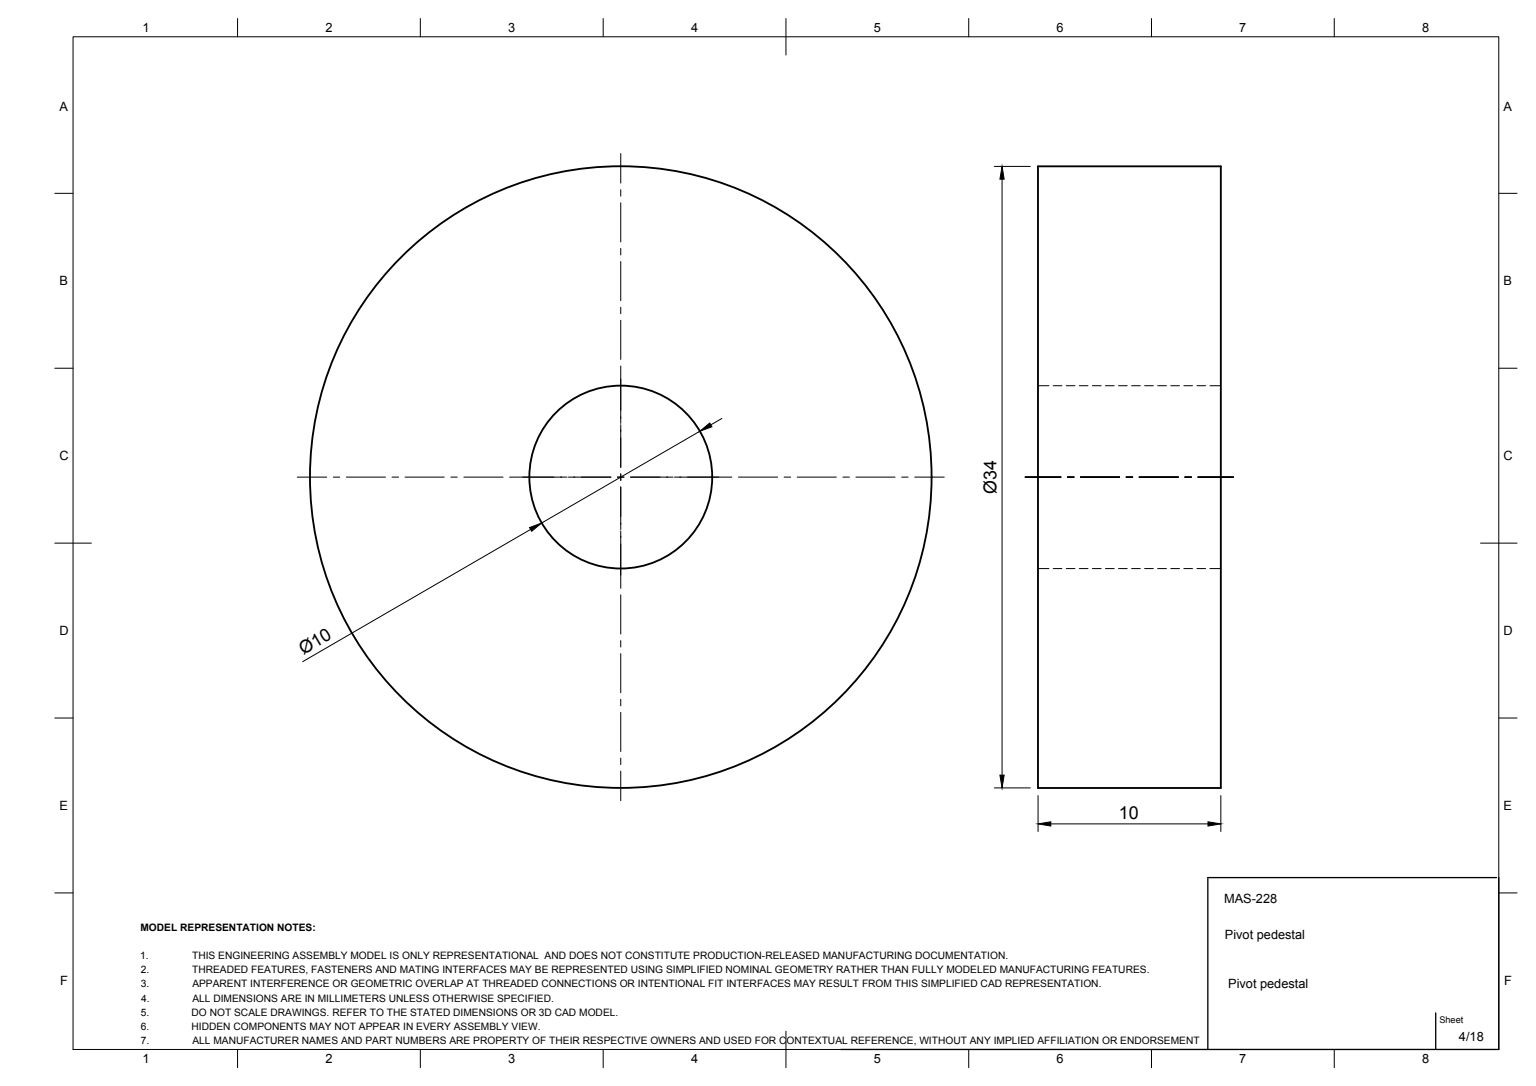
ISO-10303-21;
HEADER;
/* Generated by software containing ST-Developer
 * from STEP Tools, Inc. (www.steptools.com) 
 */

FILE_DESCRIPTION(
/* description */ ('Independent Peaucellier-Lipkin straight-line linkage. Radius arms 100
 mm, inversion-cell links 60 mm, crank radius and fixed-pivot spacing 
32 mm. Inversion constant 6400 mm squared, nominal output straight lin
e X=100 mm. Overhead bearing bridge clears the layered moving links. N
o accuracy or load rating assigned.'),
/* implementation_level */ '2;1');

FILE_NAME(
/* name */ 'Pivot pedestal.step',
/* time_stamp */ '2026-11-09T18:06:16-08:00',
/* author */ (''),
/* organization */ (''),
/* preprocessor_version */ 'ST-DEVELOPER v20.2',
/* originating_system */ 'Autodesk Translation Framework v15.17.0.0',
/* authorisation */ '');

FILE_SCHEMA (('AUTOMOTIVE_DESIGN { 1 0 10303 214 3 1 1 }'));
ENDSEC;

DATA;
#10=MECHANICAL_DESIGN_GEOMETRIC_PRESENTATION_REPRESENTATION('',(#283),#3581);
#249=SHAPE_REPRESENTATION_RELATIONSHIP('SRR','None',#3683,#266);
#266=ADVANCED_BREP_SHAPE_REPRESENTATION('',(#300),#3565);
#283=STYLED_ITEM('',(#3777),#300);
#300=MANIFOLD_SOLID_BREP('Body1',#1869);
#326=FACE_BOUND('',#560,.T.);
#327=FACE_BOUND('',#562,.T.);
#370=PLANE('',#2103);
#371=PLANE('',#2104);
#436=FACE_OUTER_BOUND('',#557,.T.);
#437=FACE_OUTER_BOUND('',#558,.T.);
#438=FACE_OUTER_BOUND('',#559,.T.);
#439=FACE_OUTER_BOUND('',#561,.T.);
#557=EDGE_LOOP('',(#1370,#1371,#1372,#1373));
#558=EDGE_LOOP('',(#1374,#1375,#1376,#1377));
#559=EDGE_LOOP('',(#1378));
#560=EDGE_LOOP('',(#1379));
#561=EDGE_LOOP('',(#1380));
#562=EDGE_LOOP('',(#1381));
#712=LINE('',#3092,#810);
#713=LINE('',#3098,#811);
#810=VECTOR('',#2428,5.);
#811=VECTOR('',#2435,12.);
#901=CIRCLE('',#2098,5.);
#902=CIRCLE('',#2099,5.);
#903=CIRCLE('',#2101,17.);
#904=CIRCLE('',#2102,17.);
#1007=VERTEX_POINT('',#3089);
#1008=VERTEX_POINT('',#3091);
#1009=VERTEX_POINT('',#3095);
#1010=VERTEX_POINT('',#3097);
#1147=EDGE_CURVE('',#1007,#1007,#901,.T.);
#1148=EDGE_CURVE('',#1007,#1008,#712,.T.);
#1149=EDGE_CURVE('',#1008,#1008,#902,.T.);
#1150=EDGE_CURVE('',#1009,#1009,#903,.F.);
#1151=EDGE_CURVE('',#1009,#1010,#713,.T.);
#1152=EDGE_CURVE('',#1010,#1010,#904,.F.);
#1370=ORIENTED_EDGE('',*,*,#1147,.F.);
#1371=ORIENTED_EDGE('',*,*,#1148,.T.);
#1372=ORIENTED_EDGE('',*,*,#1149,.T.);
#1373=ORIENTED_EDGE('',*,*,#1148,.F.);
#1374=ORIENTED_EDGE('',*,*,#1150,.F.);
#1375=ORIENTED_EDGE('',*,*,#1151,.T.);
#1376=ORIENTED_EDGE('',*,*,#1152,.T.);
#1377=ORIENTED_EDGE('',*,*,#1151,.F.);
#1378=ORIENTED_EDGE('',*,*,#1150,.T.);
#1379=ORIENTED_EDGE('',*,*,#1147,.T.);
#1380=ORIENTED_EDGE('',*,*,#1152,.F.);
#1381=ORIENTED_EDGE('',*,*,#1149,.F.);
#1713=CYLINDRICAL_SURFACE('',#2097,5.);
#1714=CYLINDRICAL_SURFACE('',#2100,17.);
#1768=ADVANCED_FACE('',(#436),#1713,.F.);
#1769=ADVANCED_FACE('',(#437),#1714,.T.);
#1770=ADVANCED_FACE('',(#438,#326),#370,.T.);
#1771=ADVANCED_FACE('',(#439,#327),#371,.F.);
#1869=CLOSED_SHELL('',(#1768,#1769,#1770,#1771));
#2096=AXIS2_PLACEMENT_3D('',#3087,#2422,#2423);
#2097=AXIS2_PLACEMENT_3D('',#3088,#2424,#2425);
#2098=AXIS2_PLACEMENT_3D('',#3090,#2426,#2427);
#2099=AXIS2_PLACEMENT_3D('',#3093,#2429,#2430);
#2100=AXIS2_PLACEMENT_3D('',#3094,#2431,#2432);
#2101=AXIS2_PLACEMENT_3D('',#3096,#2433,#2434);
#2102=AXIS2_PLACEMENT_3D('',#3099,#2436,#2437);
#2103=AXIS2_PLACEMENT_3D('',#3100,#2438,#2439);
#2104=AXIS2_PLACEMENT_3D('',#3101,#2440,#2441);
#2422=DIRECTION('axis',(0.,0.,1.));
#2423=DIRECTION('refdir',(1.,0.,0.));
#2424=DIRECTION('center_axis',(0.,0.,1.));
#2425=DIRECTION('ref_axis',(1.,0.,0.));
#2426=DIRECTION('center_axis',(0.,0.,-1.));
#2427=DIRECTION('ref_axis',(1.,0.,0.));
#2428=DIRECTION('',(0.,0.,-1.));
#2429=DIRECTION('center_axis',(0.,0.,-1.));
#2430=DIRECTION('ref_axis',(1.,0.,0.));
#2431=DIRECTION('center_axis',(0.,0.,1.));
#2432=DIRECTION('ref_axis',(1.,0.,0.));
#2433=DIRECTION('center_axis',(0.,0.,-1.));
#2434=DIRECTION('ref_axis',(1.,0.,0.));
#2435=DIRECTION('',(0.,0.,-1.));
#2436=DIRECTION('center_axis',(0.,0.,-1.));
#2437=DIRECTION('ref_axis',(1.,0.,0.));
#2438=DIRECTION('center_axis',(0.,0.,1.));
#2439=DIRECTION('ref_axis',(1.,0.,0.));
#2440=DIRECTION('center_axis',(0.,0.,1.));
#2441=DIRECTION('ref_axis',(1.,0.,0.));
#3087=CARTESIAN_POINT('',(0.,0.,0.));
#3088=CARTESIAN_POINT('Origin',(0.,0.,0.));
#3089=CARTESIAN_POINT('',(-5.,-6.12323399573677E-16,10.));
#3090=CARTESIAN_POINT('Origin',(0.,0.,10.));
#3091=CARTESIAN_POINT('',(-5.,-6.12323399573677E-16,0.));
#3092=CARTESIAN_POINT('',(-5.,-6.12323399573677E-16,0.));
#3093=CARTESIAN_POINT('Origin',(0.,0.,0.));
#3094=CARTESIAN_POINT('Origin',(0.,0.,0.));
#3095=CARTESIAN_POINT('',(-17.,2.0818995585505E-15,10.));
#3096=CARTESIAN_POINT('Origin',(0.,0.,10.));
#3097=CARTESIAN_POINT('',(-17.,2.0818995585505E-15,0.));
#3098=CARTESIAN_POINT('',(-17.,-2.0818995585505E-15,0.));
#3099=CARTESIAN_POINT('Origin',(0.,0.,0.));
#3100=CARTESIAN_POINT('Origin',(0.,0.,10.));
#3101=CARTESIAN_POINT('Origin',(0.,0.,0.));
#3546=UNCERTAINTY_MEASURE_WITH_UNIT(LENGTH_MEASURE(0.01),#3582,
'DISTANCE_ACCURACY_VALUE',
'Maximum model space distance between geometric entities at asserted c
onnectivities');
#3562=UNCERTAINTY_MEASURE_WITH_UNIT(LENGTH_MEASURE(0.01),#3582,
'DISTANCE_ACCURACY_VALUE',
'Maximum model space distance between geometric entities at asserted c
onnectivities');
#3565=(
GEOMETRIC_REPRESENTATION_CONTEXT(3)
GLOBAL_UNCERTAINTY_ASSIGNED_CONTEXT((#3546))
GLOBAL_UNIT_ASSIGNED_CONTEXT((#3582,#3584,#3585))
REPRESENTATION_CONTEXT('','3D')
);
#3581=(
GEOMETRIC_REPRESENTATION_CONTEXT(3)
GLOBAL_UNCERTAINTY_ASSIGNED_CONTEXT((#3562))
GLOBAL_UNIT_ASSIGNED_CONTEXT((#3582,#3584,#3585))
REPRESENTATION_CONTEXT('','3D')
);
#3582=(
LENGTH_UNIT()
NAMED_UNIT(*)
SI_UNIT(.MILLI.,.METRE.)
);
#3584=(
NAMED_UNIT(*)
PLANE_ANGLE_UNIT()
SI_UNIT($,.RADIAN.)
);
#3585=(
NAMED_UNIT(*)
SI_UNIT($,.STERADIAN.)
SOLID_ANGLE_UNIT()
);
#3588=SHAPE_DEFINITION_REPRESENTATION(#3606,#3683);
#3606=PRODUCT_DEFINITION_SHAPE('',$,#3702);
#3683=SHAPE_REPRESENTATION('',(#2096),#3565);
#3699=PRODUCT_DEFINITION_CONTEXT('part definition',#3755,'design');
#3702=PRODUCT_DEFINITION('Pivot pedestal','Pivot pedestal',#3720,#3699);
#3720=PRODUCT_DEFINITION_FORMATION('',$,#3759);
#3755=APPLICATION_CONTEXT(
'Core Data for Automotive Mechanical Design Process');
#3756=PRODUCT_CONTEXT('part definition',#3755,'mechanical');
#3759=PRODUCT('Pivot pedestal','Pivot pedestal','Pivot pedestal',(#3756));
#3777=PRESENTATION_STYLE_ASSIGNMENT((#3790));
#3790=SURFACE_STYLE_USAGE(.BOTH.,#3803);
#3803=SURFACE_SIDE_STYLE('',(#3816));
#3816=SURFACE_STYLE_FILL_AREA(#3829);
#3829=FILL_AREA_STYLE('Support gray',(#3842));
#3842=FILL_AREA_STYLE_COLOUR('Support gray',#3855);
#3855=COLOUR_RGB('Support gray',0.407843137254902,0.447058823529412,0.498039215686275);
ENDSEC;
END-ISO-10303-21;
